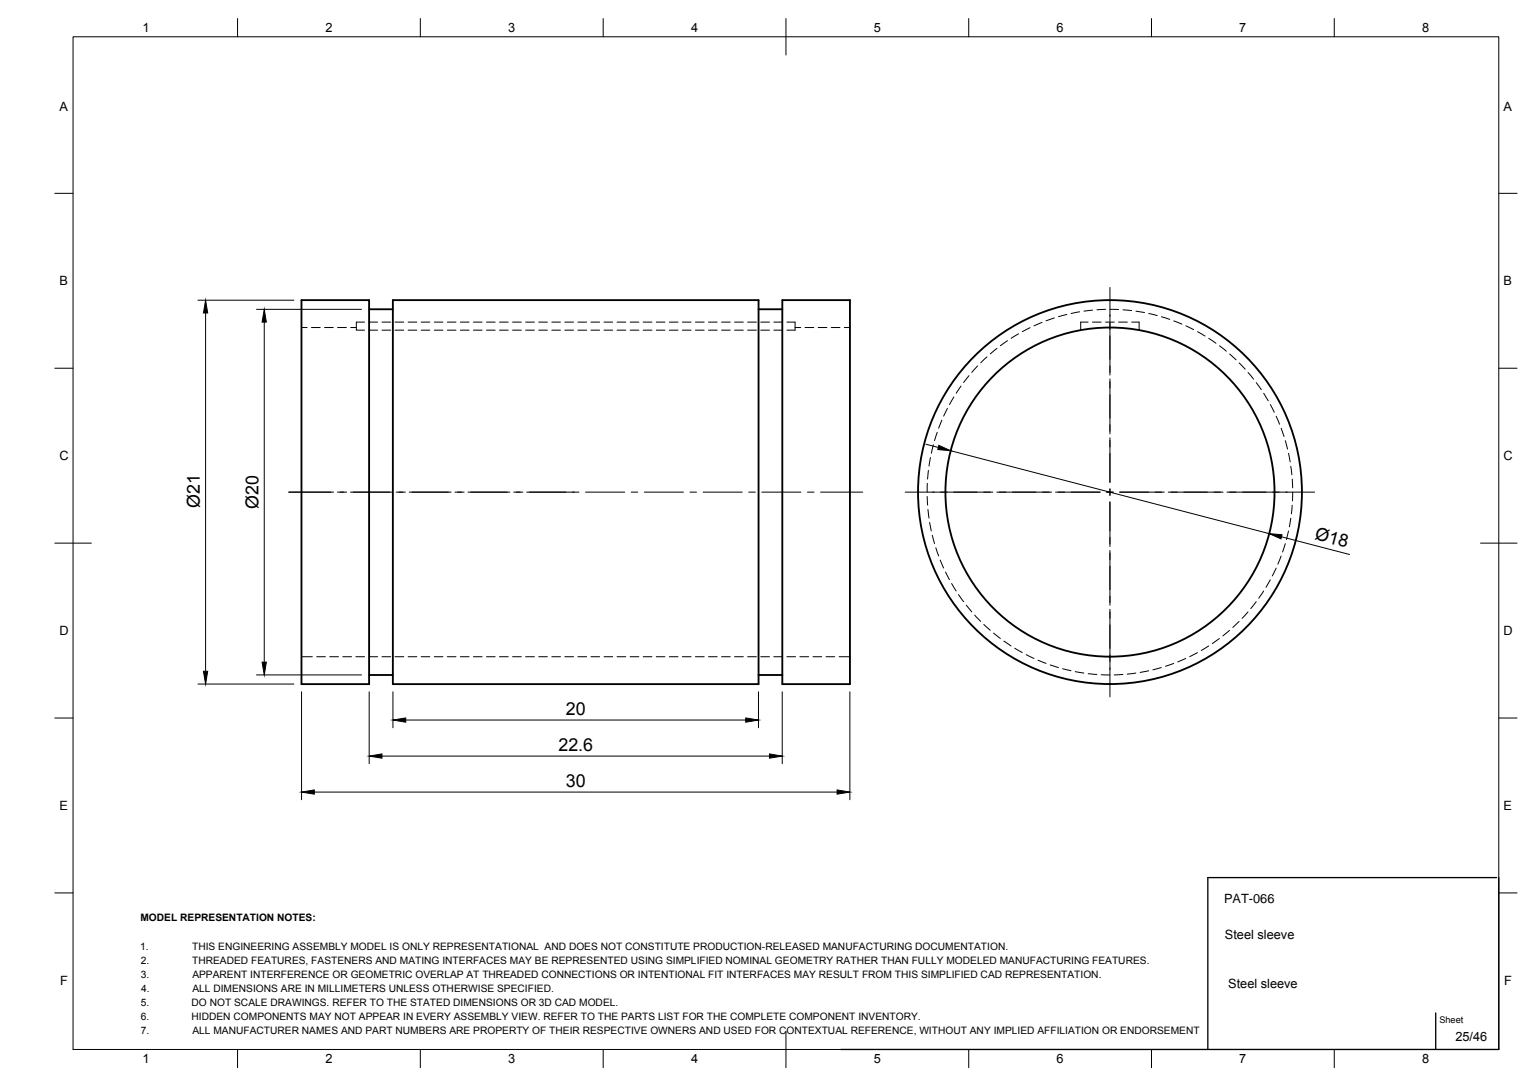
ISO-10303-21;
HEADER;
/* Generated by software containing ST-Developer
 * from STEP Tools, Inc. (www.steptools.com) 
 */

FILE_DESCRIPTION(
/* description */ ('Lever-operated bar clamp (toggle)'),
/* implementation_level */ '2;1');

FILE_NAME(
/* name */ 'Steel sleeve.step',
/* time_stamp */ '2026-10-28T03:25:02-07:00',
/* author */ (''),
/* organization */ (''),
/* preprocessor_version */ 'ST-DEVELOPER v20.2',
/* originating_system */ 'Autodesk Translation Framework v15.17.0.0',
/* authorisation */ '');

FILE_SCHEMA (('AUTOMOTIVE_DESIGN { 1 0 10303 214 3 1 1 }'));
ENDSEC;

DATA;
#10=MECHANICAL_DESIGN_GEOMETRIC_PRESENTATION_REPRESENTATION('',(#435),#12413);
#351=SHAPE_REPRESENTATION_RELATIONSHIP('SRR','None',#12592,#389);
#389=ADVANCED_BREP_SHAPE_REPRESENTATION('',(#481),#12389);
#435=STYLED_ITEM('',(#12883),#481);
#481=MANIFOLD_SOLID_BREP('Body1',#6595);
#597=FACE_BOUND('',#1599,.T.);
#598=FACE_BOUND('',#1602,.T.);
#599=FACE_BOUND('',#1605,.T.);
#600=FACE_BOUND('',#1608,.T.);
#601=FACE_BOUND('',#1611,.T.);
#602=FACE_BOUND('',#1614,.T.);
#603=FACE_BOUND('',#1616,.T.);
#756=PLANE('',#7463);
#757=PLANE('',#7465);
#758=PLANE('',#7466);
#759=PLANE('',#7468);
#760=PLANE('',#7469);
#761=PLANE('',#7470);
#762=PLANE('',#7475);
#763=PLANE('',#7479);
#764=PLANE('',#7483);
#765=PLANE('',#7487);
#766=PLANE('',#7491);
#1090=FACE_OUTER_BOUND('',#1593,.T.);
#1091=FACE_OUTER_BOUND('',#1594,.T.);
#1092=FACE_OUTER_BOUND('',#1595,.T.);
#1093=FACE_OUTER_BOUND('',#1596,.T.);
#1094=FACE_OUTER_BOUND('',#1597,.T.);
#1095=FACE_OUTER_BOUND('',#1598,.T.);
#1096=FACE_OUTER_BOUND('',#1600,.T.);
#1097=FACE_OUTER_BOUND('',#1601,.T.);
#1098=FACE_OUTER_BOUND('',#1603,.T.);
#1099=FACE_OUTER_BOUND('',#1604,.T.);
#1100=FACE_OUTER_BOUND('',#1606,.T.);
#1101=FACE_OUTER_BOUND('',#1607,.T.);
#1102=FACE_OUTER_BOUND('',#1609,.T.);
#1103=FACE_OUTER_BOUND('',#1610,.T.);
#1104=FACE_OUTER_BOUND('',#1612,.T.);
#1105=FACE_OUTER_BOUND('',#1613,.T.);
#1106=FACE_OUTER_BOUND('',#1615,.T.);
#1593=EDGE_LOOP('',(#5257,#5258,#5259,#5260));
#1594=EDGE_LOOP('',(#5261,#5262,#5263,#5264));
#1595=EDGE_LOOP('',(#5265,#5266,#5267,#5268));
#1596=EDGE_LOOP('',(#5269,#5270,#5271,#5272));
#1597=EDGE_LOOP('',(#5273,#5274,#5275,#5276));
#1598=EDGE_LOOP('',(#5277));
#1599=EDGE_LOOP('',(#5278));
#1600=EDGE_LOOP('',(#5279,#5280,#5281,#5282));
#1601=EDGE_LOOP('',(#5283));
#1602=EDGE_LOOP('',(#5284));
#1603=EDGE_LOOP('',(#5285,#5286,#5287,#5288));
#1604=EDGE_LOOP('',(#5289));
#1605=EDGE_LOOP('',(#5290));
#1606=EDGE_LOOP('',(#5291,#5292,#5293,#5294));
#1607=EDGE_LOOP('',(#5295));
#1608=EDGE_LOOP('',(#5296));
#1609=EDGE_LOOP('',(#5297,#5298,#5299,#5300));
#1610=EDGE_LOOP('',(#5301));
#1611=EDGE_LOOP('',(#5302));
#1612=EDGE_LOOP('',(#5303,#5304,#5305,#5306));
#1613=EDGE_LOOP('',(#5307));
#1614=EDGE_LOOP('',(#5308));
#1615=EDGE_LOOP('',(#5309,#5310,#5311,#5312));
#1616=EDGE_LOOP('',(#5313,#5314,#5315,#5316));
#2056=LINE('',#11322,#2497);
#2057=LINE('',#11324,#2498);
#2058=LINE('',#11325,#2499);
#2059=LINE('',#11328,#2500);
#2060=LINE('',#11330,#2501);
#2061=LINE('',#11331,#2502);
#2062=LINE('',#11336,#2503);
#2063=LINE('',#11337,#2504);
#2064=LINE('',#11339,#2505);
#2065=LINE('',#11340,#2506);
#2066=LINE('',#11350,#2507);
#2067=LINE('',#11357,#2508);
#2068=LINE('',#11364,#2509);
#2069=LINE('',#11371,#2510);
#2070=LINE('',#11378,#2511);
#2071=LINE('',#11383,#2512);
#2497=VECTOR('',#8951,1.);
#2498=VECTOR('',#8952,1.);
#2499=VECTOR('',#8953,1.);
#2500=VECTOR('',#8956,1.);
#2501=VECTOR('',#8957,1.);
#2502=VECTOR('',#8958,1.);
#2503=VECTOR('',#8963,1.);
#2504=VECTOR('',#8964,1.);
#2505=VECTOR('',#8967,1.);
#2506=VECTOR('',#8968,1.);
#2507=VECTOR('',#8981,1.05);
#2508=VECTOR('',#8990,1.);
#2509=VECTOR('',#8999,1.05);
#2510=VECTOR('',#9008,1.);
#2511=VECTOR('',#9017,1.05);
#2512=VECTOR('',#9024,0.9);
#2928=CIRCLE('',#7464,0.9);
#2929=CIRCLE('',#7467,0.9);
#2930=CIRCLE('',#7471,1.05);
#2931=CIRCLE('',#7472,0.9);
#2932=CIRCLE('',#7474,1.05);
#2933=CIRCLE('',#7476,1.);
#2934=CIRCLE('',#7478,1.);
#2935=CIRCLE('',#7480,1.05);
#2936=CIRCLE('',#7482,1.05);
#2937=CIRCLE('',#7484,1.);
#2938=CIRCLE('',#7486,1.);
#2939=CIRCLE('',#7488,1.05);
#2940=CIRCLE('',#7490,1.05);
#2941=CIRCLE('',#7492,0.9);
#3361=VERTEX_POINT('',#11318);
#3362=VERTEX_POINT('',#11319);
#3363=VERTEX_POINT('',#11321);
#3364=VERTEX_POINT('',#11323);
#3365=VERTEX_POINT('',#11327);
#3366=VERTEX_POINT('',#11329);
#3367=VERTEX_POINT('',#11333);
#3368=VERTEX_POINT('',#11335);
#3369=VERTEX_POINT('',#11343);
#3370=VERTEX_POINT('',#11345);
#3371=VERTEX_POINT('',#11348);
#3372=VERTEX_POINT('',#11352);
#3373=VERTEX_POINT('',#11355);
#3374=VERTEX_POINT('',#11359);
#3375=VERTEX_POINT('',#11362);
#3376=VERTEX_POINT('',#11366);
#3377=VERTEX_POINT('',#11369);
#3378=VERTEX_POINT('',#11373);
#3379=VERTEX_POINT('',#11376);
#3380=VERTEX_POINT('',#11380);
#4033=EDGE_CURVE('',#3361,#3362,#2928,.T.);
#4034=EDGE_CURVE('',#3363,#3361,#2056,.T.);
#4035=EDGE_CURVE('',#3364,#3363,#2057,.T.);
#4036=EDGE_CURVE('',#3362,#3364,#2058,.T.);
#4037=EDGE_CURVE('',#3362,#3365,#2059,.T.);
#4038=EDGE_CURVE('',#3366,#3364,#2060,.T.);
#4039=EDGE_CURVE('',#3366,#3365,#2061,.T.);
#4040=EDGE_CURVE('',#3365,#3367,#2929,.T.);
#4041=EDGE_CURVE('',#3368,#3366,#2062,.T.);
#4042=EDGE_CURVE('',#3367,#3368,#2063,.T.);
#4043=EDGE_CURVE('',#3367,#3361,#2064,.T.);
#4044=EDGE_CURVE('',#3368,#3363,#2065,.T.);
#4045=EDGE_CURVE('',#3369,#3369,#2930,.T.);
#4046=EDGE_CURVE('',#3370,#3370,#2931,.T.);
#4047=EDGE_CURVE('',#3371,#3371,#2932,.T.);
#4048=EDGE_CURVE('',#3371,#3369,#2066,.T.);
#4049=EDGE_CURVE('',#3372,#3372,#2933,.T.);
#4050=EDGE_CURVE('',#3373,#3373,#2934,.T.);
#4051=EDGE_CURVE('',#3373,#3372,#2067,.T.);
#4052=EDGE_CURVE('',#3374,#3374,#2935,.T.);
#4053=EDGE_CURVE('',#3375,#3375,#2936,.T.);
#4054=EDGE_CURVE('',#3375,#3374,#2068,.T.);
#4055=EDGE_CURVE('',#3376,#3376,#2937,.T.);
#4056=EDGE_CURVE('',#3377,#3377,#2938,.T.);
#4057=EDGE_CURVE('',#3377,#3376,#2069,.T.);
#4058=EDGE_CURVE('',#3378,#3378,#2939,.T.);
#4059=EDGE_CURVE('',#3379,#3379,#2940,.T.);
#4060=EDGE_CURVE('',#3379,#3378,#2070,.T.);
#4061=EDGE_CURVE('',#3380,#3380,#2941,.T.);
#4062=EDGE_CURVE('',#3380,#3370,#2071,.T.);
#5257=ORIENTED_EDGE('',*,*,#4033,.F.);
#5258=ORIENTED_EDGE('',*,*,#4034,.F.);
#5259=ORIENTED_EDGE('',*,*,#4035,.F.);
#5260=ORIENTED_EDGE('',*,*,#4036,.F.);
#5261=ORIENTED_EDGE('',*,*,#4037,.F.);
#5262=ORIENTED_EDGE('',*,*,#4036,.T.);
#5263=ORIENTED_EDGE('',*,*,#4038,.F.);
#5264=ORIENTED_EDGE('',*,*,#4039,.T.);
#5265=ORIENTED_EDGE('',*,*,#4040,.F.);
#5266=ORIENTED_EDGE('',*,*,#4039,.F.);
#5267=ORIENTED_EDGE('',*,*,#4041,.F.);
#5268=ORIENTED_EDGE('',*,*,#4042,.F.);
#5269=ORIENTED_EDGE('',*,*,#4043,.F.);
#5270=ORIENTED_EDGE('',*,*,#4042,.T.);
#5271=ORIENTED_EDGE('',*,*,#4044,.T.);
#5272=ORIENTED_EDGE('',*,*,#4034,.T.);
#5273=ORIENTED_EDGE('',*,*,#4044,.F.);
#5274=ORIENTED_EDGE('',*,*,#4041,.T.);
#5275=ORIENTED_EDGE('',*,*,#4038,.T.);
#5276=ORIENTED_EDGE('',*,*,#4035,.T.);
#5277=ORIENTED_EDGE('',*,*,#4045,.F.);
#5278=ORIENTED_EDGE('',*,*,#4046,.T.);
#5279=ORIENTED_EDGE('',*,*,#4047,.F.);
#5280=ORIENTED_EDGE('',*,*,#4048,.T.);
#5281=ORIENTED_EDGE('',*,*,#4045,.T.);
#5282=ORIENTED_EDGE('',*,*,#4048,.F.);
#5283=ORIENTED_EDGE('',*,*,#4047,.T.);
#5284=ORIENTED_EDGE('',*,*,#4049,.F.);
#5285=ORIENTED_EDGE('',*,*,#4050,.F.);
#5286=ORIENTED_EDGE('',*,*,#4051,.T.);
#5287=ORIENTED_EDGE('',*,*,#4049,.T.);
#5288=ORIENTED_EDGE('',*,*,#4051,.F.);
#5289=ORIENTED_EDGE('',*,*,#4052,.F.);
#5290=ORIENTED_EDGE('',*,*,#4050,.T.);
#5291=ORIENTED_EDGE('',*,*,#4053,.F.);
#5292=ORIENTED_EDGE('',*,*,#4054,.T.);
#5293=ORIENTED_EDGE('',*,*,#4052,.T.);
#5294=ORIENTED_EDGE('',*,*,#4054,.F.);
#5295=ORIENTED_EDGE('',*,*,#4053,.T.);
#5296=ORIENTED_EDGE('',*,*,#4055,.F.);
#5297=ORIENTED_EDGE('',*,*,#4056,.F.);
#5298=ORIENTED_EDGE('',*,*,#4057,.T.);
#5299=ORIENTED_EDGE('',*,*,#4055,.T.);
#5300=ORIENTED_EDGE('',*,*,#4057,.F.);
#5301=ORIENTED_EDGE('',*,*,#4058,.F.);
#5302=ORIENTED_EDGE('',*,*,#4056,.T.);
#5303=ORIENTED_EDGE('',*,*,#4059,.F.);
#5304=ORIENTED_EDGE('',*,*,#4060,.T.);
#5305=ORIENTED_EDGE('',*,*,#4058,.T.);
#5306=ORIENTED_EDGE('',*,*,#4060,.F.);
#5307=ORIENTED_EDGE('',*,*,#4059,.T.);
#5308=ORIENTED_EDGE('',*,*,#4061,.F.);
#5309=ORIENTED_EDGE('',*,*,#4061,.T.);
#5310=ORIENTED_EDGE('',*,*,#4062,.T.);
#5311=ORIENTED_EDGE('',*,*,#4046,.F.);
#5312=ORIENTED_EDGE('',*,*,#4062,.F.);
#5313=ORIENTED_EDGE('',*,*,#4040,.T.);
#5314=ORIENTED_EDGE('',*,*,#4043,.T.);
#5315=ORIENTED_EDGE('',*,*,#4033,.T.);
#5316=ORIENTED_EDGE('',*,*,#4037,.T.);
#6105=CYLINDRICAL_SURFACE('',#7473,1.05);
#6106=CYLINDRICAL_SURFACE('',#7477,1.);
#6107=CYLINDRICAL_SURFACE('',#7481,1.05);
#6108=CYLINDRICAL_SURFACE('',#7485,1.);
#6109=CYLINDRICAL_SURFACE('',#7489,1.05);
#6110=CYLINDRICAL_SURFACE('',#7493,0.9);
#6365=ADVANCED_FACE('',(#1090),#756,.F.);
#6366=ADVANCED_FACE('',(#1091),#757,.F.);
#6367=ADVANCED_FACE('',(#1092),#758,.F.);
#6368=ADVANCED_FACE('',(#1093),#759,.F.);
#6369=ADVANCED_FACE('',(#1094),#760,.F.);
#6370=ADVANCED_FACE('',(#1095,#597),#761,.T.);
#6371=ADVANCED_FACE('',(#1096),#6105,.T.);
#6372=ADVANCED_FACE('',(#1097,#598),#762,.T.);
#6373=ADVANCED_FACE('',(#1098),#6106,.T.);
#6374=ADVANCED_FACE('',(#1099,#599),#763,.T.);
#6375=ADVANCED_FACE('',(#1100),#6107,.T.);
#6376=ADVANCED_FACE('',(#1101,#600),#764,.T.);
#6377=ADVANCED_FACE('',(#1102),#6108,.T.);
#6378=ADVANCED_FACE('',(#1103,#601),#765,.T.);
#6379=ADVANCED_FACE('',(#1104),#6109,.T.);
#6380=ADVANCED_FACE('',(#1105,#602),#766,.T.);
#6381=ADVANCED_FACE('',(#1106,#603),#6110,.F.);
#6595=CLOSED_SHELL('',(#6365,#6366,#6367,#6368,#6369,#6370,#6371,#6372,
#6373,#6374,#6375,#6376,#6377,#6378,#6379,#6380,#6381));
#7462=AXIS2_PLACEMENT_3D('',#11316,#8945,#8946);
#7463=AXIS2_PLACEMENT_3D('',#11317,#8947,#8948);
#7464=AXIS2_PLACEMENT_3D('',#11320,#8949,#8950);
#7465=AXIS2_PLACEMENT_3D('',#11326,#8954,#8955);
#7466=AXIS2_PLACEMENT_3D('',#11332,#8959,#8960);
#7467=AXIS2_PLACEMENT_3D('',#11334,#8961,#8962);
#7468=AXIS2_PLACEMENT_3D('',#11338,#8965,#8966);
#7469=AXIS2_PLACEMENT_3D('',#11341,#8969,#8970);
#7470=AXIS2_PLACEMENT_3D('',#11342,#8971,#8972);
#7471=AXIS2_PLACEMENT_3D('',#11344,#8973,#8974);
#7472=AXIS2_PLACEMENT_3D('',#11346,#8975,#8976);
#7473=AXIS2_PLACEMENT_3D('',#11347,#8977,#8978);
#7474=AXIS2_PLACEMENT_3D('',#11349,#8979,#8980);
#7475=AXIS2_PLACEMENT_3D('',#11351,#8982,#8983);
#7476=AXIS2_PLACEMENT_3D('',#11353,#8984,#8985);
#7477=AXIS2_PLACEMENT_3D('',#11354,#8986,#8987);
#7478=AXIS2_PLACEMENT_3D('',#11356,#8988,#8989);
#7479=AXIS2_PLACEMENT_3D('',#11358,#8991,#8992);
#7480=AXIS2_PLACEMENT_3D('',#11360,#8993,#8994);
#7481=AXIS2_PLACEMENT_3D('',#11361,#8995,#8996);
#7482=AXIS2_PLACEMENT_3D('',#11363,#8997,#8998);
#7483=AXIS2_PLACEMENT_3D('',#11365,#9000,#9001);
#7484=AXIS2_PLACEMENT_3D('',#11367,#9002,#9003);
#7485=AXIS2_PLACEMENT_3D('',#11368,#9004,#9005);
#7486=AXIS2_PLACEMENT_3D('',#11370,#9006,#9007);
#7487=AXIS2_PLACEMENT_3D('',#11372,#9009,#9010);
#7488=AXIS2_PLACEMENT_3D('',#11374,#9011,#9012);
#7489=AXIS2_PLACEMENT_3D('',#11375,#9013,#9014);
#7490=AXIS2_PLACEMENT_3D('',#11377,#9015,#9016);
#7491=AXIS2_PLACEMENT_3D('',#11379,#9018,#9019);
#7492=AXIS2_PLACEMENT_3D('',#11381,#9020,#9021);
#7493=AXIS2_PLACEMENT_3D('',#11382,#9022,#9023);
#8945=DIRECTION('axis',(0.,0.,1.));
#8946=DIRECTION('refdir',(1.,0.,0.));
#8947=DIRECTION('center_axis',(0.,1.,0.));
#8948=DIRECTION('ref_axis',(0.,0.,1.));
#8949=DIRECTION('center_axis',(0.,-1.,0.));
#8950=DIRECTION('ref_axis',(1.,0.,0.));
#8951=DIRECTION('',(-1.,0.,0.));
#8952=DIRECTION('',(0.,0.,-1.));
#8953=DIRECTION('',(1.,0.,0.));
#8954=DIRECTION('center_axis',(0.,0.,1.));
#8955=DIRECTION('ref_axis',(1.,0.,0.));
#8956=DIRECTION('',(0.,-1.,0.));
#8957=DIRECTION('',(0.,1.,0.));
#8958=DIRECTION('',(-1.,0.,0.));
#8959=DIRECTION('center_axis',(0.,-1.,0.));
#8960=DIRECTION('ref_axis',(0.,0.,-1.));
#8961=DIRECTION('center_axis',(0.,1.,0.));
#8962=DIRECTION('ref_axis',(1.,0.,0.));
#8963=DIRECTION('',(0.,0.,1.));
#8964=DIRECTION('',(1.,0.,0.));
#8965=DIRECTION('center_axis',(0.,0.,-1.));
#8966=DIRECTION('ref_axis',(-1.,0.,0.));
#8967=DIRECTION('',(0.,1.,0.));
#8968=DIRECTION('',(0.,1.,0.));
#8969=DIRECTION('center_axis',(1.,0.,0.));
#8970=DIRECTION('ref_axis',(0.,0.,-1.));
#8971=DIRECTION('center_axis',(0.,1.,0.));
#8972=DIRECTION('ref_axis',(0.,0.,1.));
#8973=DIRECTION('center_axis',(0.,-1.,0.));
#8974=DIRECTION('ref_axis',(1.,0.,0.));
#8975=DIRECTION('center_axis',(0.,-1.,0.));
#8976=DIRECTION('ref_axis',(1.,0.,0.));
#8977=DIRECTION('center_axis',(0.,-1.,0.));
#8978=DIRECTION('ref_axis',(1.,0.,0.));
#8979=DIRECTION('center_axis',(0.,-1.,0.));
#8980=DIRECTION('ref_axis',(1.,0.,0.));
#8981=DIRECTION('',(0.,1.,0.));
#8982=DIRECTION('center_axis',(0.,-1.,0.));
#8983=DIRECTION('ref_axis',(0.,0.,-1.));
#8984=DIRECTION('center_axis',(0.,-1.,0.));
#8985=DIRECTION('ref_axis',(1.,0.,0.));
#8986=DIRECTION('center_axis',(0.,-1.,0.));
#8987=DIRECTION('ref_axis',(1.,0.,0.));
#8988=DIRECTION('center_axis',(0.,-1.,0.));
#8989=DIRECTION('ref_axis',(1.,0.,0.));
#8990=DIRECTION('',(0.,1.,0.));
#8991=DIRECTION('center_axis',(0.,1.,0.));
#8992=DIRECTION('ref_axis',(0.,0.,1.));
#8993=DIRECTION('center_axis',(0.,-1.,0.));
#8994=DIRECTION('ref_axis',(1.,0.,0.));
#8995=DIRECTION('center_axis',(0.,-1.,0.));
#8996=DIRECTION('ref_axis',(1.,0.,0.));
#8997=DIRECTION('center_axis',(0.,-1.,0.));
#8998=DIRECTION('ref_axis',(1.,0.,0.));
#8999=DIRECTION('',(0.,1.,0.));
#9000=DIRECTION('center_axis',(0.,-1.,0.));
#9001=DIRECTION('ref_axis',(0.,0.,-1.));
#9002=DIRECTION('center_axis',(0.,-1.,0.));
#9003=DIRECTION('ref_axis',(1.,0.,0.));
#9004=DIRECTION('center_axis',(0.,-1.,0.));
#9005=DIRECTION('ref_axis',(1.,0.,0.));
#9006=DIRECTION('center_axis',(0.,-1.,0.));
#9007=DIRECTION('ref_axis',(1.,0.,0.));
#9008=DIRECTION('',(0.,1.,0.));
#9009=DIRECTION('center_axis',(0.,1.,0.));
#9010=DIRECTION('ref_axis',(0.,0.,1.));
#9011=DIRECTION('center_axis',(0.,-1.,0.));
#9012=DIRECTION('ref_axis',(1.,0.,0.));
#9013=DIRECTION('center_axis',(0.,-1.,0.));
#9014=DIRECTION('ref_axis',(1.,0.,0.));
#9015=DIRECTION('center_axis',(0.,-1.,0.));
#9016=DIRECTION('ref_axis',(1.,0.,0.));
#9017=DIRECTION('',(0.,1.,0.));
#9018=DIRECTION('center_axis',(0.,-1.,0.));
#9019=DIRECTION('ref_axis',(0.,0.,-1.));
#9020=DIRECTION('center_axis',(0.,-1.,0.));
#9021=DIRECTION('ref_axis',(1.,0.,0.));
#9022=DIRECTION('center_axis',(0.,-1.,0.));
#9023=DIRECTION('ref_axis',(1.,0.,0.));
#9024=DIRECTION('',(0.,1.,0.));
#11316=CARTESIAN_POINT('',(0.,0.,0.));
#11317=CARTESIAN_POINT('Origin',(0.75,1.2,0.));
#11318=CARTESIAN_POINT('',(0.885663593019381,1.2,-0.16));
#11319=CARTESIAN_POINT('',(0.885663593019381,1.2,0.16));
#11320=CARTESIAN_POINT('Origin',(0.,1.2,0.));
#11321=CARTESIAN_POINT('',(0.93,1.2,-0.16));
#11322=CARTESIAN_POINT('',(0.93,1.2,-0.16));
#11323=CARTESIAN_POINT('',(0.93,1.2,0.16));
#11324=CARTESIAN_POINT('',(0.93,1.2,0.16));
#11325=CARTESIAN_POINT('',(0.57,1.2,0.16));
#11326=CARTESIAN_POINT('Origin',(0.57,0.,0.16));
#11327=CARTESIAN_POINT('',(0.885663593019381,-1.2,0.16));
#11328=CARTESIAN_POINT('',(0.885663593019381,0.,0.16));
#11329=CARTESIAN_POINT('',(0.93,-1.2,0.16));
#11330=CARTESIAN_POINT('',(0.93,0.,0.16));
#11331=CARTESIAN_POINT('',(0.57,-1.2,0.16));
#11332=CARTESIAN_POINT('Origin',(0.75,-1.2,0.));
#11333=CARTESIAN_POINT('',(0.885663593019381,-1.2,-0.16));
#11334=CARTESIAN_POINT('Origin',(0.,-1.2,0.));
#11335=CARTESIAN_POINT('',(0.93,-1.2,-0.16));
#11336=CARTESIAN_POINT('',(0.93,-1.2,0.16));
#11337=CARTESIAN_POINT('',(0.93,-1.2,-0.16));
#11338=CARTESIAN_POINT('Origin',(0.93,0.,-0.16));
#11339=CARTESIAN_POINT('',(0.885663593019381,0.,-0.16));
#11340=CARTESIAN_POINT('',(0.93,0.,-0.16));
#11341=CARTESIAN_POINT('Origin',(0.93,0.,0.16));
#11342=CARTESIAN_POINT('Origin',(1.05,1.5,0.));
#11343=CARTESIAN_POINT('',(-1.05,1.5,-1.28587913910472E-16));
#11344=CARTESIAN_POINT('Origin',(0.,1.5,0.));
#11345=CARTESIAN_POINT('',(-0.9,1.5,-1.10218211923262E-16));
#11346=CARTESIAN_POINT('Origin',(0.,1.5,0.));
#11347=CARTESIAN_POINT('Origin',(0.,1.315,0.));
#11348=CARTESIAN_POINT('',(-1.05,1.13,-1.28587913910472E-16));
#11349=CARTESIAN_POINT('Origin',(0.,1.13,0.));
#11350=CARTESIAN_POINT('',(-1.05,1.315,-1.28587913910472E-16));
#11351=CARTESIAN_POINT('Origin',(1.,1.13,0.));
#11352=CARTESIAN_POINT('',(-1.,1.13,-1.22464679914735E-16));
#11353=CARTESIAN_POINT('Origin',(0.,1.13,0.));
#11354=CARTESIAN_POINT('Origin',(0.,1.065,0.));
#11355=CARTESIAN_POINT('',(-1.,1.,-1.22464679914735E-16));
#11356=CARTESIAN_POINT('Origin',(0.,1.,0.));
#11357=CARTESIAN_POINT('',(-1.,1.065,-1.22464679914735E-16));
#11358=CARTESIAN_POINT('Origin',(1.05,1.,0.));
#11359=CARTESIAN_POINT('',(-1.05,1.,-1.28587913910472E-16));
#11360=CARTESIAN_POINT('Origin',(0.,1.,0.));
#11361=CARTESIAN_POINT('Origin',(0.,0.,0.));
#11362=CARTESIAN_POINT('',(-1.05,-1.,-1.28587913910472E-16));
#11363=CARTESIAN_POINT('Origin',(0.,-1.,0.));
#11364=CARTESIAN_POINT('',(-1.05,0.,-1.28587913910472E-16));
#11365=CARTESIAN_POINT('Origin',(1.,-1.,0.));
#11366=CARTESIAN_POINT('',(-1.,-1.,-1.22464679914735E-16));
#11367=CARTESIAN_POINT('Origin',(0.,-1.,0.));
#11368=CARTESIAN_POINT('Origin',(0.,-1.065,0.));
#11369=CARTESIAN_POINT('',(-1.,-1.13,-1.22464679914735E-16));
#11370=CARTESIAN_POINT('Origin',(0.,-1.13,0.));
#11371=CARTESIAN_POINT('',(-1.,-1.065,-1.22464679914735E-16));
#11372=CARTESIAN_POINT('Origin',(1.05,-1.13,0.));
#11373=CARTESIAN_POINT('',(-1.05,-1.13,-1.28587913910472E-16));
#11374=CARTESIAN_POINT('Origin',(0.,-1.13,0.));
#11375=CARTESIAN_POINT('Origin',(0.,-1.315,0.));
#11376=CARTESIAN_POINT('',(-1.05,-1.5,-1.28587913910472E-16));
#11377=CARTESIAN_POINT('Origin',(0.,-1.5,0.));
#11378=CARTESIAN_POINT('',(-1.05,-1.315,-1.28587913910472E-16));
#11379=CARTESIAN_POINT('Origin',(0.9,-1.5,0.));
#11380=CARTESIAN_POINT('',(-0.9,-1.5,-1.10218211923262E-16));
#11381=CARTESIAN_POINT('Origin',(0.,-1.5,0.));
#11382=CARTESIAN_POINT('Origin',(0.,0.,0.));
#11383=CARTESIAN_POINT('',(-0.9,0.,-1.10218211923262E-16));
#12343=UNCERTAINTY_MEASURE_WITH_UNIT(LENGTH_MEASURE(0.001),#12414,
'DISTANCE_ACCURACY_VALUE',
'Maximum model space distance between geometric entities at asserted c
onnectivities');
#12367=UNCERTAINTY_MEASURE_WITH_UNIT(LENGTH_MEASURE(0.001),#12414,
'DISTANCE_ACCURACY_VALUE',
'Maximum model space distance between geometric entities at asserted c
onnectivities');
#12389=(
GEOMETRIC_REPRESENTATION_CONTEXT(3)
GLOBAL_UNCERTAINTY_ASSIGNED_CONTEXT((#12343))
GLOBAL_UNIT_ASSIGNED_CONTEXT((#12414,#12416,#12417))
REPRESENTATION_CONTEXT('','3D')
);
#12413=(
GEOMETRIC_REPRESENTATION_CONTEXT(3)
GLOBAL_UNCERTAINTY_ASSIGNED_CONTEXT((#12367))
GLOBAL_UNIT_ASSIGNED_CONTEXT((#12414,#12416,#12417))
REPRESENTATION_CONTEXT('','3D')
);
#12414=(
LENGTH_UNIT()
NAMED_UNIT(*)
SI_UNIT(.CENTI.,.METRE.)
);
#12416=(
NAMED_UNIT(*)
PLANE_ANGLE_UNIT()
SI_UNIT($,.RADIAN.)
);
#12417=(
NAMED_UNIT(*)
SI_UNIT($,.STERADIAN.)
SOLID_ANGLE_UNIT()
);
#12439=SHAPE_DEFINITION_REPRESENTATION(#12489,#12592);
#12489=PRODUCT_DEFINITION_SHAPE('',$,#12638);
#12592=SHAPE_REPRESENTATION('',(#7462),#12389);
#12616=PRODUCT_DEFINITION_CONTEXT('part definition',#12753,'design');
#12638=PRODUCT_DEFINITION('Steel sleeve','Steel sleeve',#12683,#12616);
#12683=PRODUCT_DEFINITION_FORMATION('',$,#12776);
#12753=APPLICATION_CONTEXT(
'Core Data for Automotive Mechanical Design Process');
#12754=PRODUCT_CONTEXT('part definition',#12753,'mechanical');
#12776=PRODUCT('Steel sleeve','Steel sleeve','Steel sleeve',(#12754));
#12877=COLOUR_RGB('Off White',0.89,0.88,0.83);
#12878=FILL_AREA_STYLE_COLOUR('',#12877);
#12879=FILL_AREA_STYLE('',(#12878));
#12880=SURFACE_STYLE_FILL_AREA(#12879);
#12881=SURFACE_SIDE_STYLE('',(#12880));
#12882=SURFACE_STYLE_USAGE(.BOTH.,#12881);
#12883=PRESENTATION_STYLE_ASSIGNMENT((#12882));
ENDSEC;
END-ISO-10303-21;
